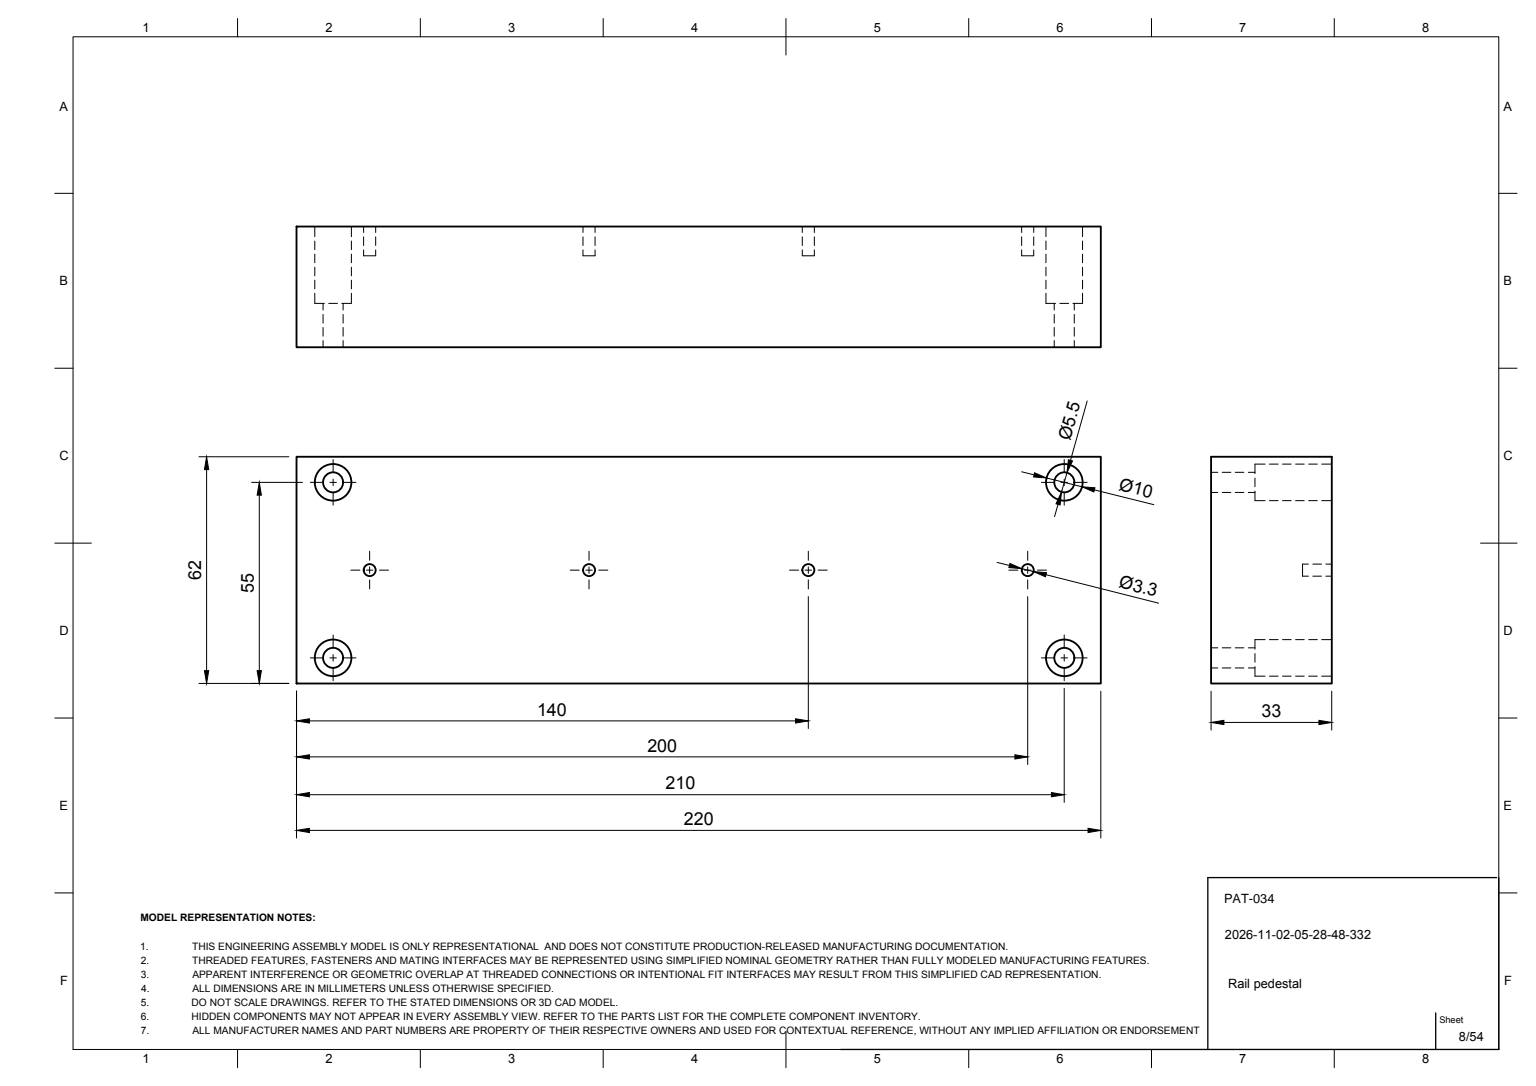
ISO-10303-21;
HEADER;
/* Generated by software containing ST-Developer
 * from STEP Tools, Inc. (www.steptools.com) 
 */

FILE_DESCRIPTION(
/* description */ ('Fatigue rig crank-slider'),
/* implementation_level */ '2;1');

FILE_NAME(
/* name */ 'Rail pedestal.step',
/* time_stamp */ '2026-10-28T03:24:50-07:00',
/* author */ (''),
/* organization */ (''),
/* preprocessor_version */ 'ST-DEVELOPER v20.2',
/* originating_system */ 'Autodesk Translation Framework v15.17.0.0',
/* authorisation */ '');

FILE_SCHEMA (('AUTOMOTIVE_DESIGN { 1 0 10303 214 3 1 1 }'));
ENDSEC;

DATA;
#10=MECHANICAL_DESIGN_GEOMETRIC_PRESENTATION_REPRESENTATION('',(#594),#16911);
#494=SHAPE_REPRESENTATION_RELATIONSHIP('SRR','None',#17133,#544);
#544=ADVANCED_BREP_SHAPE_REPRESENTATION('',(#653),#16862);
#594=STYLED_ITEM('',(#17501),#653);
#653=MANIFOLD_SOLID_BREP('Body1',#8885);
#760=FACE_BOUND('',#1888,.T.);
#761=FACE_BOUND('',#1891,.T.);
#762=FACE_BOUND('',#1894,.T.);
#763=FACE_BOUND('',#1897,.T.);
#764=FACE_BOUND('',#1907,.T.);
#765=FACE_BOUND('',#1908,.T.);
#766=FACE_BOUND('',#1909,.T.);
#767=FACE_BOUND('',#1910,.T.);
#768=FACE_BOUND('',#1911,.T.);
#769=FACE_BOUND('',#1912,.T.);
#770=FACE_BOUND('',#1913,.T.);
#771=FACE_BOUND('',#1914,.T.);
#772=FACE_BOUND('',#1916,.T.);
#773=FACE_BOUND('',#1917,.T.);
#774=FACE_BOUND('',#1918,.T.);
#775=FACE_BOUND('',#1919,.T.);
#935=PLANE('',#9664);
#936=PLANE('',#9668);
#937=PLANE('',#9672);
#938=PLANE('',#9676);
#939=PLANE('',#9680);
#940=PLANE('',#9685);
#941=PLANE('',#9690);
#942=PLANE('',#9695);
#943=PLANE('',#9705);
#944=PLANE('',#9706);
#945=PLANE('',#9707);
#946=PLANE('',#9708);
#947=PLANE('',#9709);
#948=PLANE('',#9710);
#1295=FACE_OUTER_BOUND('',#1878,.T.);
#1296=FACE_OUTER_BOUND('',#1879,.T.);
#1297=FACE_OUTER_BOUND('',#1880,.T.);
#1298=FACE_OUTER_BOUND('',#1881,.T.);
#1299=FACE_OUTER_BOUND('',#1882,.T.);
#1300=FACE_OUTER_BOUND('',#1883,.T.);
#1301=FACE_OUTER_BOUND('',#1884,.T.);
#1302=FACE_OUTER_BOUND('',#1885,.T.);
#1303=FACE_OUTER_BOUND('',#1886,.T.);
#1304=FACE_OUTER_BOUND('',#1887,.T.);
#1305=FACE_OUTER_BOUND('',#1889,.T.);
#1306=FACE_OUTER_BOUND('',#1890,.T.);
#1307=FACE_OUTER_BOUND('',#1892,.T.);
#1308=FACE_OUTER_BOUND('',#1893,.T.);
#1309=FACE_OUTER_BOUND('',#1895,.T.);
#1310=FACE_OUTER_BOUND('',#1896,.T.);
#1311=FACE_OUTER_BOUND('',#1898,.T.);
#1312=FACE_OUTER_BOUND('',#1899,.T.);
#1313=FACE_OUTER_BOUND('',#1900,.T.);
#1314=FACE_OUTER_BOUND('',#1901,.T.);
#1315=FACE_OUTER_BOUND('',#1902,.T.);
#1316=FACE_OUTER_BOUND('',#1903,.T.);
#1317=FACE_OUTER_BOUND('',#1904,.T.);
#1318=FACE_OUTER_BOUND('',#1905,.T.);
#1319=FACE_OUTER_BOUND('',#1906,.T.);
#1320=FACE_OUTER_BOUND('',#1915,.T.);
#1878=EDGE_LOOP('',(#6308,#6309,#6310,#6311));
#1879=EDGE_LOOP('',(#6312));
#1880=EDGE_LOOP('',(#6313,#6314,#6315,#6316));
#1881=EDGE_LOOP('',(#6317));
#1882=EDGE_LOOP('',(#6318,#6319,#6320,#6321));
#1883=EDGE_LOOP('',(#6322));
#1884=EDGE_LOOP('',(#6323,#6324,#6325,#6326));
#1885=EDGE_LOOP('',(#6327));
#1886=EDGE_LOOP('',(#6328,#6329,#6330,#6331));
#1887=EDGE_LOOP('',(#6332));
#1888=EDGE_LOOP('',(#6333));
#1889=EDGE_LOOP('',(#6334,#6335,#6336,#6337));
#1890=EDGE_LOOP('',(#6338));
#1891=EDGE_LOOP('',(#6339));
#1892=EDGE_LOOP('',(#6340,#6341,#6342,#6343));
#1893=EDGE_LOOP('',(#6344));
#1894=EDGE_LOOP('',(#6345));
#1895=EDGE_LOOP('',(#6346,#6347,#6348,#6349));
#1896=EDGE_LOOP('',(#6350));
#1897=EDGE_LOOP('',(#6351));
#1898=EDGE_LOOP('',(#6352,#6353,#6354,#6355));
#1899=EDGE_LOOP('',(#6356,#6357,#6358,#6359));
#1900=EDGE_LOOP('',(#6360,#6361,#6362,#6363));
#1901=EDGE_LOOP('',(#6364,#6365,#6366,#6367));
#1902=EDGE_LOOP('',(#6368,#6369,#6370,#6371));
#1903=EDGE_LOOP('',(#6372,#6373,#6374,#6375));
#1904=EDGE_LOOP('',(#6376,#6377,#6378,#6379));
#1905=EDGE_LOOP('',(#6380,#6381,#6382,#6383));
#1906=EDGE_LOOP('',(#6384,#6385,#6386,#6387));
#1907=EDGE_LOOP('',(#6388));
#1908=EDGE_LOOP('',(#6389));
#1909=EDGE_LOOP('',(#6390));
#1910=EDGE_LOOP('',(#6391));
#1911=EDGE_LOOP('',(#6392));
#1912=EDGE_LOOP('',(#6393));
#1913=EDGE_LOOP('',(#6394));
#1914=EDGE_LOOP('',(#6395));
#1915=EDGE_LOOP('',(#6396,#6397,#6398,#6399));
#1916=EDGE_LOOP('',(#6400));
#1917=EDGE_LOOP('',(#6401));
#1918=EDGE_LOOP('',(#6402));
#1919=EDGE_LOOP('',(#6403));
#2536=LINE('',#13710,#3182);
#2537=LINE('',#13717,#3183);
#2538=LINE('',#13724,#3184);
#2539=LINE('',#13731,#3185);
#2540=LINE('',#13738,#3186);
#2541=LINE('',#13747,#3187);
#2542=LINE('',#13756,#3188);
#2543=LINE('',#13765,#3189);
#2544=LINE('',#13773,#3190);
#2545=LINE('',#13777,#3191);
#2546=LINE('',#13781,#3192);
#2547=LINE('',#13785,#3193);
#2548=LINE('',#13789,#3194);
#2549=LINE('',#13791,#3195);
#2550=LINE('',#13793,#3196);
#2551=LINE('',#13794,#3197);
#2552=LINE('',#13797,#3198);
#2553=LINE('',#13799,#3199);
#2554=LINE('',#13800,#3200);
#2555=LINE('',#13803,#3201);
#2556=LINE('',#13805,#3202);
#2557=LINE('',#13806,#3203);
#2558=LINE('',#13808,#3204);
#2559=LINE('',#13809,#3205);
#3182=VECTOR('',#10982,0.164999999999999);
#3183=VECTOR('',#10991,0.164999999999999);
#3184=VECTOR('',#11000,0.165);
#3185=VECTOR('',#11009,0.164999999999999);
#3186=VECTOR('',#11018,0.5);
#3187=VECTOR('',#11029,0.5);
#3188=VECTOR('',#11040,0.5);
#3189=VECTOR('',#11051,0.5);
#3190=VECTOR('',#11062,0.274999999999999);
#3191=VECTOR('',#11067,0.275);
#3192=VECTOR('',#11072,0.275);
#3193=VECTOR('',#11077,0.274999999999999);
#3194=VECTOR('',#11080,1.);
#3195=VECTOR('',#11081,1.);
#3196=VECTOR('',#11082,1.);
#3197=VECTOR('',#11083,1.);
#3198=VECTOR('',#11086,1.);
#3199=VECTOR('',#11087,1.);
#3200=VECTOR('',#11088,1.);
#3201=VECTOR('',#11091,1.);
#3202=VECTOR('',#11092,1.);
#3203=VECTOR('',#11093,1.);
#3204=VECTOR('',#11096,1.);
#3205=VECTOR('',#11097,1.);
#3832=CIRCLE('',#9662,0.164999999999999);
#3833=CIRCLE('',#9663,0.164999999999999);
#3834=CIRCLE('',#9666,0.164999999999999);
#3835=CIRCLE('',#9667,0.164999999999999);
#3836=CIRCLE('',#9670,0.165);
#3837=CIRCLE('',#9671,0.165);
#3838=CIRCLE('',#9674,0.164999999999999);
#3839=CIRCLE('',#9675,0.164999999999999);
#3840=CIRCLE('',#9678,0.5);
#3841=CIRCLE('',#9679,0.5);
#3842=CIRCLE('',#9681,0.274999999999999);
#3843=CIRCLE('',#9683,0.5);
#3844=CIRCLE('',#9684,0.5);
#3845=CIRCLE('',#9686,0.275);
#3846=CIRCLE('',#9688,0.5);
#3847=CIRCLE('',#9689,0.5);
#3848=CIRCLE('',#9691,0.275);
#3849=CIRCLE('',#9693,0.5);
#3850=CIRCLE('',#9694,0.5);
#3851=CIRCLE('',#9696,0.274999999999999);
#3852=CIRCLE('',#9698,0.274999999999999);
#3853=CIRCLE('',#9700,0.275);
#3854=CIRCLE('',#9702,0.275);
#3855=CIRCLE('',#9704,0.274999999999999);
#4256=VERTEX_POINT('',#13707);
#4257=VERTEX_POINT('',#13709);
#4258=VERTEX_POINT('',#13714);
#4259=VERTEX_POINT('',#13716);
#4260=VERTEX_POINT('',#13721);
#4261=VERTEX_POINT('',#13723);
#4262=VERTEX_POINT('',#13728);
#4263=VERTEX_POINT('',#13730);
#4264=VERTEX_POINT('',#13735);
#4265=VERTEX_POINT('',#13737);
#4266=VERTEX_POINT('',#13741);
#4267=VERTEX_POINT('',#13744);
#4268=VERTEX_POINT('',#13746);
#4269=VERTEX_POINT('',#13750);
#4270=VERTEX_POINT('',#13753);
#4271=VERTEX_POINT('',#13755);
#4272=VERTEX_POINT('',#13759);
#4273=VERTEX_POINT('',#13762);
#4274=VERTEX_POINT('',#13764);
#4275=VERTEX_POINT('',#13768);
#4276=VERTEX_POINT('',#13771);
#4277=VERTEX_POINT('',#13775);
#4278=VERTEX_POINT('',#13779);
#4279=VERTEX_POINT('',#13783);
#4280=VERTEX_POINT('',#13787);
#4281=VERTEX_POINT('',#13788);
#4282=VERTEX_POINT('',#13790);
#4283=VERTEX_POINT('',#13792);
#4284=VERTEX_POINT('',#13796);
#4285=VERTEX_POINT('',#13798);
#4286=VERTEX_POINT('',#13802);
#4287=VERTEX_POINT('',#13804);
#5052=EDGE_CURVE('',#4256,#4256,#3832,.T.);
#5053=EDGE_CURVE('',#4256,#4257,#2536,.T.);
#5054=EDGE_CURVE('',#4257,#4257,#3833,.T.);
#5055=EDGE_CURVE('',#4258,#4258,#3834,.T.);
#5056=EDGE_CURVE('',#4258,#4259,#2537,.T.);
#5057=EDGE_CURVE('',#4259,#4259,#3835,.T.);
#5058=EDGE_CURVE('',#4260,#4260,#3836,.T.);
#5059=EDGE_CURVE('',#4260,#4261,#2538,.T.);
#5060=EDGE_CURVE('',#4261,#4261,#3837,.T.);
#5061=EDGE_CURVE('',#4262,#4262,#3838,.T.);
#5062=EDGE_CURVE('',#4262,#4263,#2539,.T.);
#5063=EDGE_CURVE('',#4263,#4263,#3839,.T.);
#5064=EDGE_CURVE('',#4264,#4264,#3840,.T.);
#5065=EDGE_CURVE('',#4264,#4265,#2540,.T.);
#5066=EDGE_CURVE('',#4265,#4265,#3841,.T.);
#5067=EDGE_CURVE('',#4266,#4266,#3842,.T.);
#5068=EDGE_CURVE('',#4267,#4267,#3843,.T.);
#5069=EDGE_CURVE('',#4267,#4268,#2541,.T.);
#5070=EDGE_CURVE('',#4268,#4268,#3844,.T.);
#5071=EDGE_CURVE('',#4269,#4269,#3845,.T.);
#5072=EDGE_CURVE('',#4270,#4270,#3846,.T.);
#5073=EDGE_CURVE('',#4270,#4271,#2542,.T.);
#5074=EDGE_CURVE('',#4271,#4271,#3847,.T.);
#5075=EDGE_CURVE('',#4272,#4272,#3848,.T.);
#5076=EDGE_CURVE('',#4273,#4273,#3849,.T.);
#5077=EDGE_CURVE('',#4273,#4274,#2543,.T.);
#5078=EDGE_CURVE('',#4274,#4274,#3850,.T.);
#5079=EDGE_CURVE('',#4275,#4275,#3851,.T.);
#5080=EDGE_CURVE('',#4276,#4276,#3852,.T.);
#5081=EDGE_CURVE('',#4276,#4266,#2544,.T.);
#5082=EDGE_CURVE('',#4277,#4277,#3853,.T.);
#5083=EDGE_CURVE('',#4277,#4269,#2545,.T.);
#5084=EDGE_CURVE('',#4278,#4278,#3854,.T.);
#5085=EDGE_CURVE('',#4278,#4272,#2546,.T.);
#5086=EDGE_CURVE('',#4279,#4279,#3855,.T.);
#5087=EDGE_CURVE('',#4279,#4275,#2547,.T.);
#5088=EDGE_CURVE('',#4280,#4281,#2548,.T.);
#5089=EDGE_CURVE('',#4281,#4282,#2549,.T.);
#5090=EDGE_CURVE('',#4283,#4282,#2550,.T.);
#5091=EDGE_CURVE('',#4280,#4283,#2551,.T.);
#5092=EDGE_CURVE('',#4284,#4280,#2552,.T.);
#5093=EDGE_CURVE('',#4285,#4283,#2553,.T.);
#5094=EDGE_CURVE('',#4284,#4285,#2554,.T.);
#5095=EDGE_CURVE('',#4286,#4284,#2555,.T.);
#5096=EDGE_CURVE('',#4287,#4285,#2556,.T.);
#5097=EDGE_CURVE('',#4286,#4287,#2557,.T.);
#5098=EDGE_CURVE('',#4281,#4286,#2558,.T.);
#5099=EDGE_CURVE('',#4282,#4287,#2559,.T.);
#6308=ORIENTED_EDGE('',*,*,#5052,.F.);
#6309=ORIENTED_EDGE('',*,*,#5053,.T.);
#6310=ORIENTED_EDGE('',*,*,#5054,.F.);
#6311=ORIENTED_EDGE('',*,*,#5053,.F.);
#6312=ORIENTED_EDGE('',*,*,#5052,.T.);
#6313=ORIENTED_EDGE('',*,*,#5055,.F.);
#6314=ORIENTED_EDGE('',*,*,#5056,.T.);
#6315=ORIENTED_EDGE('',*,*,#5057,.F.);
#6316=ORIENTED_EDGE('',*,*,#5056,.F.);
#6317=ORIENTED_EDGE('',*,*,#5055,.T.);
#6318=ORIENTED_EDGE('',*,*,#5058,.F.);
#6319=ORIENTED_EDGE('',*,*,#5059,.T.);
#6320=ORIENTED_EDGE('',*,*,#5060,.F.);
#6321=ORIENTED_EDGE('',*,*,#5059,.F.);
#6322=ORIENTED_EDGE('',*,*,#5058,.T.);
#6323=ORIENTED_EDGE('',*,*,#5061,.F.);
#6324=ORIENTED_EDGE('',*,*,#5062,.T.);
#6325=ORIENTED_EDGE('',*,*,#5063,.F.);
#6326=ORIENTED_EDGE('',*,*,#5062,.F.);
#6327=ORIENTED_EDGE('',*,*,#5061,.T.);
#6328=ORIENTED_EDGE('',*,*,#5064,.F.);
#6329=ORIENTED_EDGE('',*,*,#5065,.T.);
#6330=ORIENTED_EDGE('',*,*,#5066,.F.);
#6331=ORIENTED_EDGE('',*,*,#5065,.F.);
#6332=ORIENTED_EDGE('',*,*,#5064,.T.);
#6333=ORIENTED_EDGE('',*,*,#5067,.F.);
#6334=ORIENTED_EDGE('',*,*,#5068,.F.);
#6335=ORIENTED_EDGE('',*,*,#5069,.T.);
#6336=ORIENTED_EDGE('',*,*,#5070,.F.);
#6337=ORIENTED_EDGE('',*,*,#5069,.F.);
#6338=ORIENTED_EDGE('',*,*,#5068,.T.);
#6339=ORIENTED_EDGE('',*,*,#5071,.F.);
#6340=ORIENTED_EDGE('',*,*,#5072,.F.);
#6341=ORIENTED_EDGE('',*,*,#5073,.T.);
#6342=ORIENTED_EDGE('',*,*,#5074,.F.);
#6343=ORIENTED_EDGE('',*,*,#5073,.F.);
#6344=ORIENTED_EDGE('',*,*,#5072,.T.);
#6345=ORIENTED_EDGE('',*,*,#5075,.F.);
#6346=ORIENTED_EDGE('',*,*,#5076,.F.);
#6347=ORIENTED_EDGE('',*,*,#5077,.T.);
#6348=ORIENTED_EDGE('',*,*,#5078,.F.);
#6349=ORIENTED_EDGE('',*,*,#5077,.F.);
#6350=ORIENTED_EDGE('',*,*,#5076,.T.);
#6351=ORIENTED_EDGE('',*,*,#5079,.F.);
#6352=ORIENTED_EDGE('',*,*,#5080,.F.);
#6353=ORIENTED_EDGE('',*,*,#5081,.T.);
#6354=ORIENTED_EDGE('',*,*,#5067,.T.);
#6355=ORIENTED_EDGE('',*,*,#5081,.F.);
#6356=ORIENTED_EDGE('',*,*,#5082,.F.);
#6357=ORIENTED_EDGE('',*,*,#5083,.T.);
#6358=ORIENTED_EDGE('',*,*,#5071,.T.);
#6359=ORIENTED_EDGE('',*,*,#5083,.F.);
#6360=ORIENTED_EDGE('',*,*,#5084,.F.);
#6361=ORIENTED_EDGE('',*,*,#5085,.T.);
#6362=ORIENTED_EDGE('',*,*,#5075,.T.);
#6363=ORIENTED_EDGE('',*,*,#5085,.F.);
#6364=ORIENTED_EDGE('',*,*,#5086,.F.);
#6365=ORIENTED_EDGE('',*,*,#5087,.T.);
#6366=ORIENTED_EDGE('',*,*,#5079,.T.);
#6367=ORIENTED_EDGE('',*,*,#5087,.F.);
#6368=ORIENTED_EDGE('',*,*,#5088,.T.);
#6369=ORIENTED_EDGE('',*,*,#5089,.T.);
#6370=ORIENTED_EDGE('',*,*,#5090,.F.);
#6371=ORIENTED_EDGE('',*,*,#5091,.F.);
#6372=ORIENTED_EDGE('',*,*,#5092,.T.);
#6373=ORIENTED_EDGE('',*,*,#5091,.T.);
#6374=ORIENTED_EDGE('',*,*,#5093,.F.);
#6375=ORIENTED_EDGE('',*,*,#5094,.F.);
#6376=ORIENTED_EDGE('',*,*,#5095,.T.);
#6377=ORIENTED_EDGE('',*,*,#5094,.T.);
#6378=ORIENTED_EDGE('',*,*,#5096,.F.);
#6379=ORIENTED_EDGE('',*,*,#5097,.F.);
#6380=ORIENTED_EDGE('',*,*,#5098,.T.);
#6381=ORIENTED_EDGE('',*,*,#5097,.T.);
#6382=ORIENTED_EDGE('',*,*,#5099,.F.);
#6383=ORIENTED_EDGE('',*,*,#5089,.F.);
#6384=ORIENTED_EDGE('',*,*,#5099,.T.);
#6385=ORIENTED_EDGE('',*,*,#5096,.T.);
#6386=ORIENTED_EDGE('',*,*,#5093,.T.);
#6387=ORIENTED_EDGE('',*,*,#5090,.T.);
#6388=ORIENTED_EDGE('',*,*,#5066,.T.);
#6389=ORIENTED_EDGE('',*,*,#5070,.T.);
#6390=ORIENTED_EDGE('',*,*,#5074,.T.);
#6391=ORIENTED_EDGE('',*,*,#5078,.T.);
#6392=ORIENTED_EDGE('',*,*,#5063,.T.);
#6393=ORIENTED_EDGE('',*,*,#5060,.T.);
#6394=ORIENTED_EDGE('',*,*,#5057,.T.);
#6395=ORIENTED_EDGE('',*,*,#5054,.T.);
#6396=ORIENTED_EDGE('',*,*,#5098,.F.);
#6397=ORIENTED_EDGE('',*,*,#5088,.F.);
#6398=ORIENTED_EDGE('',*,*,#5092,.F.);
#6399=ORIENTED_EDGE('',*,*,#5095,.F.);
#6400=ORIENTED_EDGE('',*,*,#5080,.T.);
#6401=ORIENTED_EDGE('',*,*,#5082,.T.);
#6402=ORIENTED_EDGE('',*,*,#5084,.T.);
#6403=ORIENTED_EDGE('',*,*,#5086,.T.);
#8236=CYLINDRICAL_SURFACE('',#9661,0.164999999999999);
#8237=CYLINDRICAL_SURFACE('',#9665,0.164999999999999);
#8238=CYLINDRICAL_SURFACE('',#9669,0.165);
#8239=CYLINDRICAL_SURFACE('',#9673,0.164999999999999);
#8240=CYLINDRICAL_SURFACE('',#9677,0.5);
#8241=CYLINDRICAL_SURFACE('',#9682,0.5);
#8242=CYLINDRICAL_SURFACE('',#9687,0.5);
#8243=CYLINDRICAL_SURFACE('',#9692,0.5);
#8244=CYLINDRICAL_SURFACE('',#9697,0.274999999999999);
#8245=CYLINDRICAL_SURFACE('',#9699,0.275);
#8246=CYLINDRICAL_SURFACE('',#9701,0.275);
#8247=CYLINDRICAL_SURFACE('',#9703,0.274999999999999);
#8433=ADVANCED_FACE('',(#1295),#8236,.F.);
#8434=ADVANCED_FACE('',(#1296),#935,.T.);
#8435=ADVANCED_FACE('',(#1297),#8237,.F.);
#8436=ADVANCED_FACE('',(#1298),#936,.T.);
#8437=ADVANCED_FACE('',(#1299),#8238,.F.);
#8438=ADVANCED_FACE('',(#1300),#937,.T.);
#8439=ADVANCED_FACE('',(#1301),#8239,.F.);
#8440=ADVANCED_FACE('',(#1302),#938,.T.);
#8441=ADVANCED_FACE('',(#1303),#8240,.F.);
#8442=ADVANCED_FACE('',(#1304,#760),#939,.T.);
#8443=ADVANCED_FACE('',(#1305),#8241,.F.);
#8444=ADVANCED_FACE('',(#1306,#761),#940,.T.);
#8445=ADVANCED_FACE('',(#1307),#8242,.F.);
#8446=ADVANCED_FACE('',(#1308,#762),#941,.T.);
#8447=ADVANCED_FACE('',(#1309),#8243,.F.);
#8448=ADVANCED_FACE('',(#1310,#763),#942,.T.);
#8449=ADVANCED_FACE('',(#1311),#8244,.F.);
#8450=ADVANCED_FACE('',(#1312),#8245,.F.);
#8451=ADVANCED_FACE('',(#1313),#8246,.F.);
#8452=ADVANCED_FACE('',(#1314),#8247,.F.);
#8453=ADVANCED_FACE('',(#1315),#943,.T.);
#8454=ADVANCED_FACE('',(#1316),#944,.T.);
#8455=ADVANCED_FACE('',(#1317),#945,.T.);
#8456=ADVANCED_FACE('',(#1318),#946,.T.);
#8457=ADVANCED_FACE('',(#1319,#764,#765,#766,#767,#768,#769,#770,#771),
#947,.T.);
#8458=ADVANCED_FACE('',(#1320,#772,#773,#774,#775),#948,.F.);
#8885=CLOSED_SHELL('',(#8433,#8434,#8435,#8436,#8437,#8438,#8439,#8440,
#8441,#8442,#8443,#8444,#8445,#8446,#8447,#8448,#8449,#8450,#8451,#8452,
#8453,#8454,#8455,#8456,#8457,#8458));
#9660=AXIS2_PLACEMENT_3D('',#13705,#10976,#10977);
#9661=AXIS2_PLACEMENT_3D('',#13706,#10978,#10979);
#9662=AXIS2_PLACEMENT_3D('',#13708,#10980,#10981);
#9663=AXIS2_PLACEMENT_3D('',#13711,#10983,#10984);
#9664=AXIS2_PLACEMENT_3D('',#13712,#10985,#10986);
#9665=AXIS2_PLACEMENT_3D('',#13713,#10987,#10988);
#9666=AXIS2_PLACEMENT_3D('',#13715,#10989,#10990);
#9667=AXIS2_PLACEMENT_3D('',#13718,#10992,#10993);
#9668=AXIS2_PLACEMENT_3D('',#13719,#10994,#10995);
#9669=AXIS2_PLACEMENT_3D('',#13720,#10996,#10997);
#9670=AXIS2_PLACEMENT_3D('',#13722,#10998,#10999);
#9671=AXIS2_PLACEMENT_3D('',#13725,#11001,#11002);
#9672=AXIS2_PLACEMENT_3D('',#13726,#11003,#11004);
#9673=AXIS2_PLACEMENT_3D('',#13727,#11005,#11006);
#9674=AXIS2_PLACEMENT_3D('',#13729,#11007,#11008);
#9675=AXIS2_PLACEMENT_3D('',#13732,#11010,#11011);
#9676=AXIS2_PLACEMENT_3D('',#13733,#11012,#11013);
#9677=AXIS2_PLACEMENT_3D('',#13734,#11014,#11015);
#9678=AXIS2_PLACEMENT_3D('',#13736,#11016,#11017);
#9679=AXIS2_PLACEMENT_3D('',#13739,#11019,#11020);
#9680=AXIS2_PLACEMENT_3D('',#13740,#11021,#11022);
#9681=AXIS2_PLACEMENT_3D('',#13742,#11023,#11024);
#9682=AXIS2_PLACEMENT_3D('',#13743,#11025,#11026);
#9683=AXIS2_PLACEMENT_3D('',#13745,#11027,#11028);
#9684=AXIS2_PLACEMENT_3D('',#13748,#11030,#11031);
#9685=AXIS2_PLACEMENT_3D('',#13749,#11032,#11033);
#9686=AXIS2_PLACEMENT_3D('',#13751,#11034,#11035);
#9687=AXIS2_PLACEMENT_3D('',#13752,#11036,#11037);
#9688=AXIS2_PLACEMENT_3D('',#13754,#11038,#11039);
#9689=AXIS2_PLACEMENT_3D('',#13757,#11041,#11042);
#9690=AXIS2_PLACEMENT_3D('',#13758,#11043,#11044);
#9691=AXIS2_PLACEMENT_3D('',#13760,#11045,#11046);
#9692=AXIS2_PLACEMENT_3D('',#13761,#11047,#11048);
#9693=AXIS2_PLACEMENT_3D('',#13763,#11049,#11050);
#9694=AXIS2_PLACEMENT_3D('',#13766,#11052,#11053);
#9695=AXIS2_PLACEMENT_3D('',#13767,#11054,#11055);
#9696=AXIS2_PLACEMENT_3D('',#13769,#11056,#11057);
#9697=AXIS2_PLACEMENT_3D('',#13770,#11058,#11059);
#9698=AXIS2_PLACEMENT_3D('',#13772,#11060,#11061);
#9699=AXIS2_PLACEMENT_3D('',#13774,#11063,#11064);
#9700=AXIS2_PLACEMENT_3D('',#13776,#11065,#11066);
#9701=AXIS2_PLACEMENT_3D('',#13778,#11068,#11069);
#9702=AXIS2_PLACEMENT_3D('',#13780,#11070,#11071);
#9703=AXIS2_PLACEMENT_3D('',#13782,#11073,#11074);
#9704=AXIS2_PLACEMENT_3D('',#13784,#11075,#11076);
#9705=AXIS2_PLACEMENT_3D('',#13786,#11078,#11079);
#9706=AXIS2_PLACEMENT_3D('',#13795,#11084,#11085);
#9707=AXIS2_PLACEMENT_3D('',#13801,#11089,#11090);
#9708=AXIS2_PLACEMENT_3D('',#13807,#11094,#11095);
#9709=AXIS2_PLACEMENT_3D('',#13810,#11098,#11099);
#9710=AXIS2_PLACEMENT_3D('',#13811,#11100,#11101);
#10976=DIRECTION('axis',(0.,0.,1.));
#10977=DIRECTION('refdir',(1.,0.,0.));
#10978=DIRECTION('center_axis',(0.,0.,1.));
#10979=DIRECTION('ref_axis',(1.,0.,0.));
#10980=DIRECTION('center_axis',(0.,0.,1.));
#10981=DIRECTION('ref_axis',(1.,0.,0.));
#10982=DIRECTION('',(0.,0.,1.));
#10983=DIRECTION('center_axis',(0.,0.,-1.));
#10984=DIRECTION('ref_axis',(1.,0.,0.));
#10985=DIRECTION('center_axis',(0.,0.,1.));
#10986=DIRECTION('ref_axis',(1.,0.,0.));
#10987=DIRECTION('center_axis',(0.,0.,1.));
#10988=DIRECTION('ref_axis',(1.,0.,0.));
#10989=DIRECTION('center_axis',(0.,0.,1.));
#10990=DIRECTION('ref_axis',(1.,0.,0.));
#10991=DIRECTION('',(0.,0.,1.));
#10992=DIRECTION('center_axis',(0.,0.,-1.));
#10993=DIRECTION('ref_axis',(1.,0.,0.));
#10994=DIRECTION('center_axis',(0.,0.,1.));
#10995=DIRECTION('ref_axis',(1.,0.,0.));
#10996=DIRECTION('center_axis',(0.,0.,1.));
#10997=DIRECTION('ref_axis',(1.,0.,0.));
#10998=DIRECTION('center_axis',(0.,0.,1.));
#10999=DIRECTION('ref_axis',(1.,0.,0.));
#11000=DIRECTION('',(0.,0.,1.));
#11001=DIRECTION('center_axis',(0.,0.,-1.));
#11002=DIRECTION('ref_axis',(1.,0.,0.));
#11003=DIRECTION('center_axis',(0.,0.,1.));
#11004=DIRECTION('ref_axis',(1.,0.,0.));
#11005=DIRECTION('center_axis',(0.,0.,1.));
#11006=DIRECTION('ref_axis',(1.,0.,0.));
#11007=DIRECTION('center_axis',(0.,0.,1.));
#11008=DIRECTION('ref_axis',(1.,0.,0.));
#11009=DIRECTION('',(0.,0.,1.));
#11010=DIRECTION('center_axis',(0.,0.,-1.));
#11011=DIRECTION('ref_axis',(1.,0.,0.));
#11012=DIRECTION('center_axis',(0.,0.,1.));
#11013=DIRECTION('ref_axis',(1.,0.,0.));
#11014=DIRECTION('center_axis',(0.,0.,1.));
#11015=DIRECTION('ref_axis',(1.,0.,0.));
#11016=DIRECTION('center_axis',(0.,0.,1.));
#11017=DIRECTION('ref_axis',(1.,0.,0.));
#11018=DIRECTION('',(0.,0.,1.));
#11019=DIRECTION('center_axis',(0.,0.,-1.));
#11020=DIRECTION('ref_axis',(1.,0.,0.));
#11021=DIRECTION('center_axis',(0.,0.,1.));
#11022=DIRECTION('ref_axis',(1.,0.,0.));
#11023=DIRECTION('center_axis',(0.,0.,1.));
#11024=DIRECTION('ref_axis',(1.,0.,0.));
#11025=DIRECTION('center_axis',(0.,0.,1.));
#11026=DIRECTION('ref_axis',(1.,0.,0.));
#11027=DIRECTION('center_axis',(0.,0.,1.));
#11028=DIRECTION('ref_axis',(1.,0.,0.));
#11029=DIRECTION('',(0.,0.,1.));
#11030=DIRECTION('center_axis',(0.,0.,-1.));
#11031=DIRECTION('ref_axis',(1.,0.,0.));
#11032=DIRECTION('center_axis',(0.,0.,1.));
#11033=DIRECTION('ref_axis',(1.,0.,0.));
#11034=DIRECTION('center_axis',(0.,0.,1.));
#11035=DIRECTION('ref_axis',(1.,0.,0.));
#11036=DIRECTION('center_axis',(0.,0.,1.));
#11037=DIRECTION('ref_axis',(1.,0.,0.));
#11038=DIRECTION('center_axis',(0.,0.,1.));
#11039=DIRECTION('ref_axis',(1.,0.,0.));
#11040=DIRECTION('',(0.,0.,1.));
#11041=DIRECTION('center_axis',(0.,0.,-1.));
#11042=DIRECTION('ref_axis',(1.,0.,0.));
#11043=DIRECTION('center_axis',(0.,0.,1.));
#11044=DIRECTION('ref_axis',(1.,0.,0.));
#11045=DIRECTION('center_axis',(0.,0.,1.));
#11046=DIRECTION('ref_axis',(1.,0.,0.));
#11047=DIRECTION('center_axis',(0.,0.,1.));
#11048=DIRECTION('ref_axis',(1.,0.,0.));
#11049=DIRECTION('center_axis',(0.,0.,1.));
#11050=DIRECTION('ref_axis',(1.,0.,0.));
#11051=DIRECTION('',(0.,0.,1.));
#11052=DIRECTION('center_axis',(0.,0.,-1.));
#11053=DIRECTION('ref_axis',(1.,0.,0.));
#11054=DIRECTION('center_axis',(0.,0.,1.));
#11055=DIRECTION('ref_axis',(1.,0.,0.));
#11056=DIRECTION('center_axis',(0.,0.,1.));
#11057=DIRECTION('ref_axis',(1.,0.,0.));
#11058=DIRECTION('center_axis',(0.,0.,1.));
#11059=DIRECTION('ref_axis',(1.,0.,0.));
#11060=DIRECTION('center_axis',(0.,0.,1.));
#11061=DIRECTION('ref_axis',(1.,0.,0.));
#11062=DIRECTION('',(0.,0.,1.));
#11063=DIRECTION('center_axis',(0.,0.,1.));
#11064=DIRECTION('ref_axis',(1.,0.,0.));
#11065=DIRECTION('center_axis',(0.,0.,1.));
#11066=DIRECTION('ref_axis',(1.,0.,0.));
#11067=DIRECTION('',(0.,0.,1.));
#11068=DIRECTION('center_axis',(0.,0.,1.));
#11069=DIRECTION('ref_axis',(1.,0.,0.));
#11070=DIRECTION('center_axis',(0.,0.,1.));
#11071=DIRECTION('ref_axis',(1.,0.,0.));
#11072=DIRECTION('',(0.,0.,1.));
#11073=DIRECTION('center_axis',(0.,0.,1.));
#11074=DIRECTION('ref_axis',(1.,0.,0.));
#11075=DIRECTION('center_axis',(0.,0.,1.));
#11076=DIRECTION('ref_axis',(1.,0.,0.));
#11077=DIRECTION('',(0.,0.,1.));
#11078=DIRECTION('center_axis',(0.,1.,0.));
#11079=DIRECTION('ref_axis',(-1.,0.,0.));
#11080=DIRECTION('',(-1.,0.,0.));
#11081=DIRECTION('',(0.,0.,1.));
#11082=DIRECTION('',(-1.,0.,0.));
#11083=DIRECTION('',(0.,0.,1.));
#11084=DIRECTION('center_axis',(1.,0.,0.));
#11085=DIRECTION('ref_axis',(0.,1.,0.));
#11086=DIRECTION('',(0.,1.,0.));
#11087=DIRECTION('',(0.,1.,0.));
#11088=DIRECTION('',(0.,0.,1.));
#11089=DIRECTION('center_axis',(0.,-1.,0.));
#11090=DIRECTION('ref_axis',(1.,0.,0.));
#11091=DIRECTION('',(1.,0.,0.));
#11092=DIRECTION('',(1.,0.,0.));
#11093=DIRECTION('',(0.,0.,1.));
#11094=DIRECTION('center_axis',(-1.,0.,0.));
#11095=DIRECTION('ref_axis',(0.,-1.,0.));
#11096=DIRECTION('',(0.,-1.,0.));
#11097=DIRECTION('',(0.,-1.,0.));
#11098=DIRECTION('center_axis',(0.,0.,1.));
#11099=DIRECTION('ref_axis',(1.,0.,0.));
#11100=DIRECTION('center_axis',(0.,0.,1.));
#11101=DIRECTION('ref_axis',(1.,0.,0.));
#13705=CARTESIAN_POINT('',(0.,0.,0.));
#13706=CARTESIAN_POINT('Origin',(16.,0.,3.5));
#13707=CARTESIAN_POINT('',(15.835,-2.02066721859312E-17,3.5));
#13708=CARTESIAN_POINT('Origin',(16.,0.,3.5));
#13709=CARTESIAN_POINT('',(15.835,2.02066721859312E-17,4.3));
#13710=CARTESIAN_POINT('',(15.835,-2.02066721859312E-17,3.5));
#13711=CARTESIAN_POINT('Origin',(16.,0.,4.3));
#13712=CARTESIAN_POINT('Origin',(16.,0.,3.5));
#13713=CARTESIAN_POINT('Origin',(10.,0.,3.5));
#13714=CARTESIAN_POINT('',(9.835,-2.02066721859312E-17,3.5));
#13715=CARTESIAN_POINT('Origin',(10.,0.,3.5));
#13716=CARTESIAN_POINT('',(9.835,2.02066721859312E-17,4.3));
#13717=CARTESIAN_POINT('',(9.835,-2.02066721859312E-17,3.5));
#13718=CARTESIAN_POINT('Origin',(10.,0.,4.3));
#13719=CARTESIAN_POINT('Origin',(10.,0.,3.5));
#13720=CARTESIAN_POINT('Origin',(4.,0.,3.5));
#13721=CARTESIAN_POINT('',(3.835,-2.02066721859313E-17,3.5));
#13722=CARTESIAN_POINT('Origin',(4.,0.,3.5));
#13723=CARTESIAN_POINT('',(3.835,2.02066721859313E-17,4.3));
#13724=CARTESIAN_POINT('',(3.835,-2.02066721859313E-17,3.5));
#13725=CARTESIAN_POINT('Origin',(4.,0.,4.3));
#13726=CARTESIAN_POINT('Origin',(4.,0.,3.5));
#13727=CARTESIAN_POINT('Origin',(22.,0.,3.5));
#13728=CARTESIAN_POINT('',(21.835,-2.02066721859312E-17,3.5));
#13729=CARTESIAN_POINT('Origin',(22.,0.,3.5));
#13730=CARTESIAN_POINT('',(21.835,2.02066721859312E-17,4.3));
#13731=CARTESIAN_POINT('',(21.835,-2.02066721859312E-17,3.5));
#13732=CARTESIAN_POINT('Origin',(22.,0.,4.3));
#13733=CARTESIAN_POINT('Origin',(22.,0.,3.5));
#13734=CARTESIAN_POINT('Origin',(23.,-2.4,2.2));
#13735=CARTESIAN_POINT('',(22.5,-2.4,2.2));
#13736=CARTESIAN_POINT('Origin',(23.,-2.4,2.2));
#13737=CARTESIAN_POINT('',(22.5,-2.4,4.3));
#13738=CARTESIAN_POINT('',(22.5,-2.4,2.2));
#13739=CARTESIAN_POINT('Origin',(23.,-2.4,4.3));
#13740=CARTESIAN_POINT('Origin',(23.,-2.4,2.2));
#13741=CARTESIAN_POINT('',(22.725,-2.4,2.2));
#13742=CARTESIAN_POINT('Origin',(23.,-2.4,2.2));
#13743=CARTESIAN_POINT('Origin',(3.,2.4,2.2));
#13744=CARTESIAN_POINT('',(2.5,2.4,2.2));
#13745=CARTESIAN_POINT('Origin',(3.,2.4,2.2));
#13746=CARTESIAN_POINT('',(2.5,2.4,4.3));
#13747=CARTESIAN_POINT('',(2.5,2.4,2.2));
#13748=CARTESIAN_POINT('Origin',(3.,2.4,4.3));
#13749=CARTESIAN_POINT('Origin',(3.,2.4,2.2));
#13750=CARTESIAN_POINT('',(2.725,2.4,2.2));
#13751=CARTESIAN_POINT('Origin',(3.,2.4,2.2));
#13752=CARTESIAN_POINT('Origin',(3.,-2.4,2.2));
#13753=CARTESIAN_POINT('',(2.5,-2.4,2.2));
#13754=CARTESIAN_POINT('Origin',(3.,-2.4,2.2));
#13755=CARTESIAN_POINT('',(2.5,-2.4,4.3));
#13756=CARTESIAN_POINT('',(2.5,-2.4,2.2));
#13757=CARTESIAN_POINT('Origin',(3.,-2.4,4.3));
#13758=CARTESIAN_POINT('Origin',(3.,-2.4,2.2));
#13759=CARTESIAN_POINT('',(2.725,-2.4,2.2));
#13760=CARTESIAN_POINT('Origin',(3.,-2.4,2.2));
#13761=CARTESIAN_POINT('Origin',(23.,2.4,2.2));
#13762=CARTESIAN_POINT('',(22.5,2.4,2.2));
#13763=CARTESIAN_POINT('Origin',(23.,2.4,2.2));
#13764=CARTESIAN_POINT('',(22.5,2.4,4.3));
#13765=CARTESIAN_POINT('',(22.5,2.4,2.2));
#13766=CARTESIAN_POINT('Origin',(23.,2.4,4.3));
#13767=CARTESIAN_POINT('Origin',(23.,2.4,2.2));
#13768=CARTESIAN_POINT('',(22.725,2.4,2.2));
#13769=CARTESIAN_POINT('Origin',(23.,2.4,2.2));
#13770=CARTESIAN_POINT('Origin',(23.,-2.4,0.9));
#13771=CARTESIAN_POINT('',(22.725,-2.4,1.));
#13772=CARTESIAN_POINT('Origin',(23.,-2.4,1.));
#13773=CARTESIAN_POINT('',(22.725,-2.4,0.9));
#13774=CARTESIAN_POINT('Origin',(3.,2.4,0.9));
#13775=CARTESIAN_POINT('',(2.725,2.4,1.));
#13776=CARTESIAN_POINT('Origin',(3.,2.4,1.));
#13777=CARTESIAN_POINT('',(2.725,2.4,0.9));
#13778=CARTESIAN_POINT('Origin',(3.,-2.4,0.9));
#13779=CARTESIAN_POINT('',(2.725,-2.4,1.));
#13780=CARTESIAN_POINT('Origin',(3.,-2.4,1.));
#13781=CARTESIAN_POINT('',(2.725,-2.4,0.9));
#13782=CARTESIAN_POINT('Origin',(23.,2.4,0.9));
#13783=CARTESIAN_POINT('',(22.725,2.4,1.));
#13784=CARTESIAN_POINT('Origin',(23.,2.4,1.));
#13785=CARTESIAN_POINT('',(22.725,2.4,0.9));
#13786=CARTESIAN_POINT('Origin',(24.,3.1,1.));
#13787=CARTESIAN_POINT('',(24.,3.1,1.));
#13788=CARTESIAN_POINT('',(2.,3.1,1.));
#13789=CARTESIAN_POINT('',(24.,3.1,1.));
#13790=CARTESIAN_POINT('',(2.,3.1,4.3));
#13791=CARTESIAN_POINT('',(2.,3.1,1.));
#13792=CARTESIAN_POINT('',(24.,3.1,4.3));
#13793=CARTESIAN_POINT('',(24.,3.1,4.3));
#13794=CARTESIAN_POINT('',(24.,3.1,1.));
#13795=CARTESIAN_POINT('Origin',(24.,-3.1,1.));
#13796=CARTESIAN_POINT('',(24.,-3.1,1.));
#13797=CARTESIAN_POINT('',(24.,-3.1,1.));
#13798=CARTESIAN_POINT('',(24.,-3.1,4.3));
#13799=CARTESIAN_POINT('',(24.,-3.1,4.3));
#13800=CARTESIAN_POINT('',(24.,-3.1,1.));
#13801=CARTESIAN_POINT('Origin',(2.,-3.1,1.));
#13802=CARTESIAN_POINT('',(2.,-3.1,1.));
#13803=CARTESIAN_POINT('',(2.,-3.1,1.));
#13804=CARTESIAN_POINT('',(2.,-3.1,4.3));
#13805=CARTESIAN_POINT('',(2.,-3.1,4.3));
#13806=CARTESIAN_POINT('',(2.,-3.1,1.));
#13807=CARTESIAN_POINT('Origin',(2.,3.1,1.));
#13808=CARTESIAN_POINT('',(2.,3.1,1.));
#13809=CARTESIAN_POINT('',(2.,3.1,4.3));
#13810=CARTESIAN_POINT('Origin',(13.,0.,4.3));
#13811=CARTESIAN_POINT('Origin',(13.,0.,1.));
#16803=UNCERTAINTY_MEASURE_WITH_UNIT(LENGTH_MEASURE(0.001),#16912,
'DISTANCE_ACCURACY_VALUE',
'Maximum model space distance between geometric entities at asserted c
onnectivities');
#16852=UNCERTAINTY_MEASURE_WITH_UNIT(LENGTH_MEASURE(0.001),#16912,
'DISTANCE_ACCURACY_VALUE',
'Maximum model space distance between geometric entities at asserted c
onnectivities');
#16862=(
GEOMETRIC_REPRESENTATION_CONTEXT(3)
GLOBAL_UNCERTAINTY_ASSIGNED_CONTEXT((#16803))
GLOBAL_UNIT_ASSIGNED_CONTEXT((#16912,#16914,#16915))
REPRESENTATION_CONTEXT('','3D')
);
#16911=(
GEOMETRIC_REPRESENTATION_CONTEXT(3)
GLOBAL_UNCERTAINTY_ASSIGNED_CONTEXT((#16852))
GLOBAL_UNIT_ASSIGNED_CONTEXT((#16912,#16914,#16915))
REPRESENTATION_CONTEXT('','3D')
);
#16912=(
LENGTH_UNIT()
NAMED_UNIT(*)
SI_UNIT(.CENTI.,.METRE.)
);
#16914=(
NAMED_UNIT(*)
PLANE_ANGLE_UNIT()
SI_UNIT($,.RADIAN.)
);
#16915=(
NAMED_UNIT(*)
SI_UNIT($,.STERADIAN.)
SOLID_ANGLE_UNIT()
);
#16925=SHAPE_DEFINITION_REPRESENTATION(#16983,#17133);
#16983=PRODUCT_DEFINITION_SHAPE('',$,#17192);
#17133=SHAPE_REPRESENTATION('',(#9660),#16862);
#17182=PRODUCT_DEFINITION_CONTEXT('part definition',#17358,'design');
#17192=PRODUCT_DEFINITION('Rail pedestal','Rail pedestal',#17250,#17182);
#17250=PRODUCT_DEFINITION_FORMATION('',$,#17369);
#17358=APPLICATION_CONTEXT(
'Core Data for Automotive Mechanical Design Process');
#17359=PRODUCT_CONTEXT('part definition',#17358,'mechanical');
#17369=PRODUCT('Rail pedestal','Rail pedestal','Rail pedestal',(#17359));
#17495=COLOUR_RGB('Off White',0.89,0.88,0.83);
#17496=FILL_AREA_STYLE_COLOUR('',#17495);
#17497=FILL_AREA_STYLE('',(#17496));
#17498=SURFACE_STYLE_FILL_AREA(#17497);
#17499=SURFACE_SIDE_STYLE('',(#17498));
#17500=SURFACE_STYLE_USAGE(.BOTH.,#17499);
#17501=PRESENTATION_STYLE_ASSIGNMENT((#17500));
ENDSEC;
END-ISO-10303-21;
